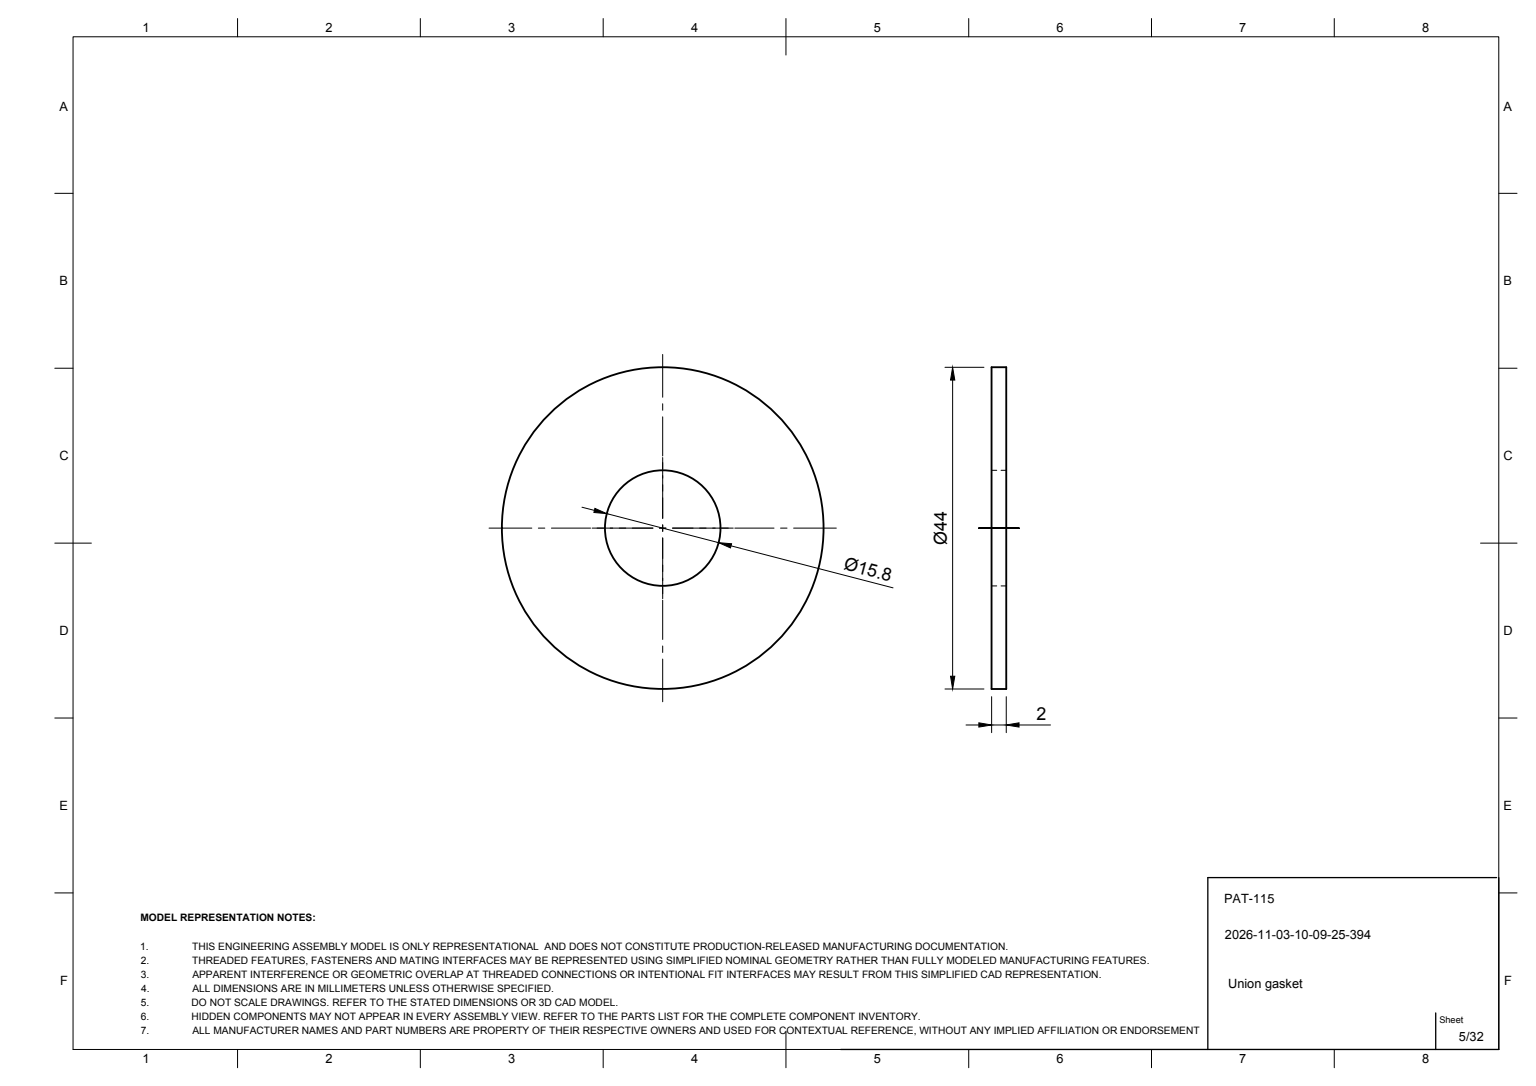
ISO-10303-21;
HEADER;
/* Generated by software containing ST-Developer
 * from STEP Tools, Inc. (www.steptools.com) 
 */

FILE_DESCRIPTION(
/* description */ ('Union bypass pipe loop'),
/* implementation_level */ '2;1');

FILE_NAME(
/* name */ 'Union gasket.step',
/* time_stamp */ '2026-10-27T21:00:29-07:00',
/* author */ (''),
/* organization */ (''),
/* preprocessor_version */ 'ST-DEVELOPER v20.2',
/* originating_system */ 'Autodesk Translation Framework v15.17.0.0',
/* authorisation */ '');

FILE_SCHEMA (('AUTOMOTIVE_DESIGN { 1 0 10303 214 3 1 1 }'));
ENDSEC;

DATA;
#10=MECHANICAL_DESIGN_GEOMETRIC_PRESENTATION_REPRESENTATION('',(#459),#10095);
#395=SHAPE_REPRESENTATION_RELATIONSHIP('SRR','None',#10264,#427);
#427=ADVANCED_BREP_SHAPE_REPRESENTATION('',(#489),#10076);
#459=STYLED_ITEM('',(#10486),#489);
#489=MANIFOLD_SOLID_BREP('Body1',#5532);
#577=FACE_BOUND('',#1385,.T.);
#578=FACE_BOUND('',#1387,.T.);
#721=PLANE('',#6230);
#722=PLANE('',#6231);
#984=FACE_OUTER_BOUND('',#1382,.T.);
#985=FACE_OUTER_BOUND('',#1383,.T.);
#986=FACE_OUTER_BOUND('',#1384,.T.);
#987=FACE_OUTER_BOUND('',#1386,.T.);
#1382=EDGE_LOOP('',(#4340,#4341,#4342,#4343));
#1383=EDGE_LOOP('',(#4344,#4345,#4346,#4347));
#1384=EDGE_LOOP('',(#4348));
#1385=EDGE_LOOP('',(#4349));
#1386=EDGE_LOOP('',(#4350));
#1387=EDGE_LOOP('',(#4351));
#1795=LINE('',#9152,#2171);
#1796=LINE('',#9158,#2172);
#2171=VECTOR('',#7433,0.79);
#2172=VECTOR('',#7440,2.2);
#2492=CIRCLE('',#6225,0.79);
#2493=CIRCLE('',#6226,0.79);
#2494=CIRCLE('',#6228,2.2);
#2495=CIRCLE('',#6229,2.2);
#2828=VERTEX_POINT('',#9149);
#2829=VERTEX_POINT('',#9151);
#2830=VERTEX_POINT('',#9155);
#2831=VERTEX_POINT('',#9157);
#3368=EDGE_CURVE('',#2828,#2828,#2492,.T.);
#3369=EDGE_CURVE('',#2828,#2829,#1795,.T.);
#3370=EDGE_CURVE('',#2829,#2829,#2493,.T.);
#3371=EDGE_CURVE('',#2830,#2830,#2494,.T.);
#3372=EDGE_CURVE('',#2830,#2831,#1796,.T.);
#3373=EDGE_CURVE('',#2831,#2831,#2495,.T.);
#4340=ORIENTED_EDGE('',*,*,#3368,.F.);
#4341=ORIENTED_EDGE('',*,*,#3369,.T.);
#4342=ORIENTED_EDGE('',*,*,#3370,.T.);
#4343=ORIENTED_EDGE('',*,*,#3369,.F.);
#4344=ORIENTED_EDGE('',*,*,#3371,.F.);
#4345=ORIENTED_EDGE('',*,*,#3372,.T.);
#4346=ORIENTED_EDGE('',*,*,#3373,.T.);
#4347=ORIENTED_EDGE('',*,*,#3372,.F.);
#4348=ORIENTED_EDGE('',*,*,#3371,.T.);
#4349=ORIENTED_EDGE('',*,*,#3368,.T.);
#4350=ORIENTED_EDGE('',*,*,#3373,.F.);
#4351=ORIENTED_EDGE('',*,*,#3370,.F.);
#5129=CYLINDRICAL_SURFACE('',#6224,0.79);
#5130=CYLINDRICAL_SURFACE('',#6227,2.2);
#5333=ADVANCED_FACE('',(#984),#5129,.F.);
#5334=ADVANCED_FACE('',(#985),#5130,.T.);
#5335=ADVANCED_FACE('',(#986,#577),#721,.T.);
#5336=ADVANCED_FACE('',(#987,#578),#722,.F.);
#5532=CLOSED_SHELL('',(#5333,#5334,#5335,#5336));
#6223=AXIS2_PLACEMENT_3D('',#9147,#7427,#7428);
#6224=AXIS2_PLACEMENT_3D('',#9148,#7429,#7430);
#6225=AXIS2_PLACEMENT_3D('',#9150,#7431,#7432);
#6226=AXIS2_PLACEMENT_3D('',#9153,#7434,#7435);
#6227=AXIS2_PLACEMENT_3D('',#9154,#7436,#7437);
#6228=AXIS2_PLACEMENT_3D('',#9156,#7438,#7439);
#6229=AXIS2_PLACEMENT_3D('',#9159,#7441,#7442);
#6230=AXIS2_PLACEMENT_3D('',#9160,#7443,#7444);
#6231=AXIS2_PLACEMENT_3D('',#9161,#7445,#7446);
#7427=DIRECTION('axis',(0.,0.,1.));
#7428=DIRECTION('refdir',(1.,0.,0.));
#7429=DIRECTION('center_axis',(1.,0.,0.));
#7430=DIRECTION('ref_axis',(0.,0.,-1.));
#7431=DIRECTION('center_axis',(-1.,0.,0.));
#7432=DIRECTION('ref_axis',(0.,0.,-1.));
#7433=DIRECTION('',(-1.,0.,0.));
#7434=DIRECTION('center_axis',(-1.,0.,0.));
#7435=DIRECTION('ref_axis',(0.,0.,-1.));
#7436=DIRECTION('center_axis',(1.,0.,0.));
#7437=DIRECTION('ref_axis',(0.,0.,-1.));
#7438=DIRECTION('center_axis',(1.,0.,0.));
#7439=DIRECTION('ref_axis',(0.,0.,-1.));
#7440=DIRECTION('',(-1.,0.,0.));
#7441=DIRECTION('center_axis',(1.,0.,0.));
#7442=DIRECTION('ref_axis',(0.,0.,-1.));
#7443=DIRECTION('center_axis',(1.,0.,0.));
#7444=DIRECTION('ref_axis',(0.,0.,-1.));
#7445=DIRECTION('center_axis',(1.,0.,0.));
#7446=DIRECTION('ref_axis',(0.,0.,-1.));
#9147=CARTESIAN_POINT('',(0.,0.,0.));
#9148=CARTESIAN_POINT('Origin',(-0.1,0.,6.));
#9149=CARTESIAN_POINT('',(0.1,-9.67470971326409E-17,6.79));
#9150=CARTESIAN_POINT('Origin',(0.1,0.,6.));
#9151=CARTESIAN_POINT('',(-0.1,-9.67470971326409E-17,6.79));
#9152=CARTESIAN_POINT('',(-0.1,-9.67470971326409E-17,6.79));
#9153=CARTESIAN_POINT('Origin',(-0.1,0.,6.));
#9154=CARTESIAN_POINT('Origin',(-0.1,0.,6.));
#9155=CARTESIAN_POINT('',(0.1,-2.69422295812418E-16,8.2));
#9156=CARTESIAN_POINT('Origin',(0.1,0.,6.));
#9157=CARTESIAN_POINT('',(-0.1,-2.69422295812418E-16,8.2));
#9158=CARTESIAN_POINT('',(-0.1,-2.69422295812418E-16,8.2));
#9159=CARTESIAN_POINT('Origin',(-0.1,0.,6.));
#9160=CARTESIAN_POINT('Origin',(0.1,0.,6.));
#9161=CARTESIAN_POINT('Origin',(-0.1,0.,6.));
#10039=UNCERTAINTY_MEASURE_WITH_UNIT(LENGTH_MEASURE(0.001),#10096,
'DISTANCE_ACCURACY_VALUE',
'Maximum model space distance between geometric entities at asserted c
onnectivities');
#10058=UNCERTAINTY_MEASURE_WITH_UNIT(LENGTH_MEASURE(0.001),#10096,
'DISTANCE_ACCURACY_VALUE',
'Maximum model space distance between geometric entities at asserted c
onnectivities');
#10076=(
GEOMETRIC_REPRESENTATION_CONTEXT(3)
GLOBAL_UNCERTAINTY_ASSIGNED_CONTEXT((#10039))
GLOBAL_UNIT_ASSIGNED_CONTEXT((#10096,#10098,#10099))
REPRESENTATION_CONTEXT('','3D')
);
#10095=(
GEOMETRIC_REPRESENTATION_CONTEXT(3)
GLOBAL_UNCERTAINTY_ASSIGNED_CONTEXT((#10058))
GLOBAL_UNIT_ASSIGNED_CONTEXT((#10096,#10098,#10099))
REPRESENTATION_CONTEXT('','3D')
);
#10096=(
LENGTH_UNIT()
NAMED_UNIT(*)
SI_UNIT(.CENTI.,.METRE.)
);
#10098=(
NAMED_UNIT(*)
PLANE_ANGLE_UNIT()
SI_UNIT($,.RADIAN.)
);
#10099=(
NAMED_UNIT(*)
SI_UNIT($,.STERADIAN.)
SOLID_ANGLE_UNIT()
);
#10117=SHAPE_DEFINITION_REPRESENTATION(#10188,#10264);
#10188=PRODUCT_DEFINITION_SHAPE('',$,#10301);
#10264=SHAPE_REPRESENTATION('',(#6223),#10076);
#10283=PRODUCT_DEFINITION_CONTEXT('part definition',#10393,'design');
#10301=PRODUCT_DEFINITION('Union gasket','Union gasket',#10337,#10283);
#10337=PRODUCT_DEFINITION_FORMATION('',$,#10412);
#10393=APPLICATION_CONTEXT(
'Core Data for Automotive Mechanical Design Process');
#10394=PRODUCT_CONTEXT('part definition',#10393,'mechanical');
#10412=PRODUCT('Union gasket','Union gasket','Union gasket',(#10394));
#10480=COLOUR_RGB('Light Blue',0.38,0.62,0.78);
#10481=FILL_AREA_STYLE_COLOUR('',#10480);
#10482=FILL_AREA_STYLE('',(#10481));
#10483=SURFACE_STYLE_FILL_AREA(#10482);
#10484=SURFACE_SIDE_STYLE('',(#10483));
#10485=SURFACE_STYLE_USAGE(.BOTH.,#10484);
#10486=PRESENTATION_STYLE_ASSIGNMENT((#10485));
ENDSEC;
END-ISO-10303-21;
